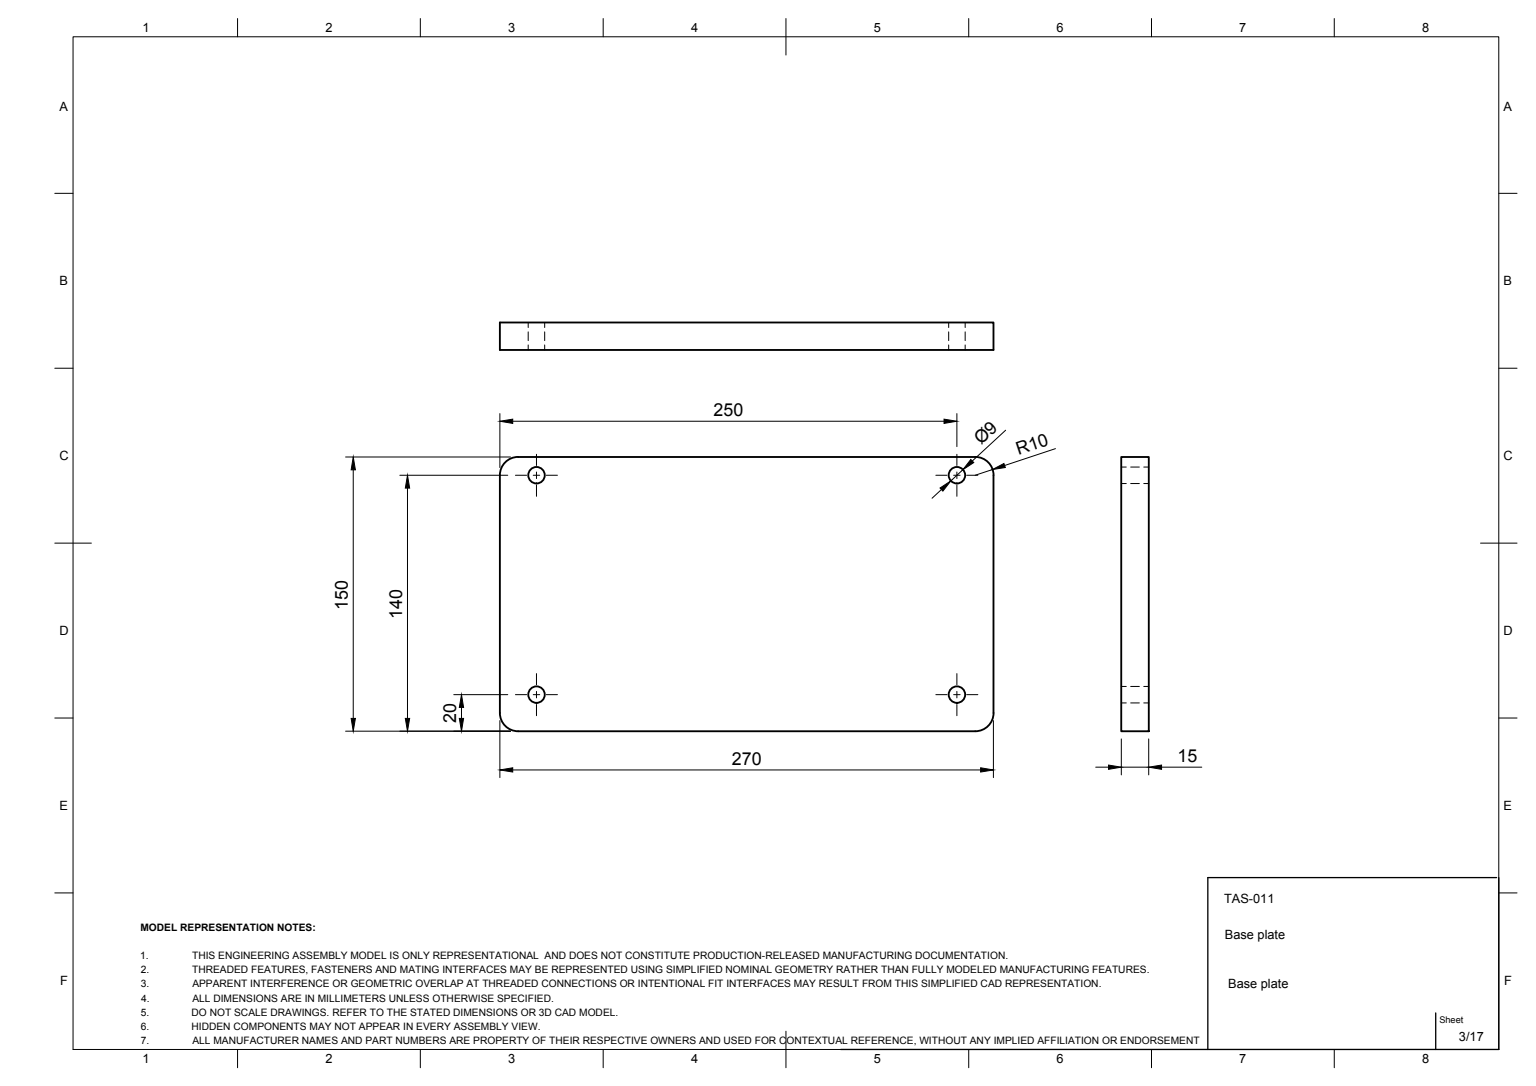
ISO-10303-21;
HEADER;
/* Generated by software containing ST-Developer
 * from STEP Tools, Inc. (www.steptools.com) 
 */

FILE_DESCRIPTION(
/* description */ (
'Independent manual bench leaf bending machine,200mm work width. Fabri
cated welded frame and folding leaf, repeated bushed and fully retaine
d hinge hardware, two handles with bonded grips, beveled clamping beam
 and modeledM12 clamp screws.2mm omitted-workpiece assembly reference 
gap, not a capacity claim. Native135deg hinge travel. Weld sizing, pro
duction fits, material condition, bending capacity, strength and life 
unassigned.'),
/* implementation_level */ '2;1');

FILE_NAME(
/* name */ 'Base plate.step',
/* time_stamp */ '2026-11-14T09:11:34-08:00',
/* author */ (''),
/* organization */ (''),
/* preprocessor_version */ 'ST-DEVELOPER v20.2',
/* originating_system */ 'Autodesk Translation Framework v15.17.0.0',
/* authorisation */ '');

FILE_SCHEMA (('AUTOMOTIVE_DESIGN { 1 0 10303 214 3 1 1 }'));
ENDSEC;

DATA;
#10=MECHANICAL_DESIGN_GEOMETRIC_PRESENTATION_REPRESENTATION('',(#446),#37701);
#410=SHAPE_REPRESENTATION_RELATIONSHIP('SRR','None',#37779,#428);
#428=ADVANCED_BREP_SHAPE_REPRESENTATION('',(#464),#37683);
#446=STYLED_ITEM('',(#37878),#464);
#464=MANIFOLD_SOLID_BREP('Body1',#4144);
#482=FACE_BOUND('',#817,.T.);
#483=FACE_BOUND('',#818,.T.);
#484=FACE_BOUND('',#819,.T.);
#485=FACE_BOUND('',#820,.T.);
#486=FACE_BOUND('',#832,.T.);
#487=FACE_BOUND('',#833,.T.);
#488=FACE_BOUND('',#834,.T.);
#489=FACE_BOUND('',#835,.T.);
#516=PLANE('',#4366);
#517=PLANE('',#4367);
#518=PLANE('',#4377);
#519=PLANE('',#4380);
#520=PLANE('',#4391);
#521=PLANE('',#4392);
#602=FACE_OUTER_BOUND('',#814,.T.);
#603=FACE_OUTER_BOUND('',#815,.T.);
#604=FACE_OUTER_BOUND('',#816,.T.);
#605=FACE_OUTER_BOUND('',#821,.T.);
#606=FACE_OUTER_BOUND('',#822,.T.);
#607=FACE_OUTER_BOUND('',#823,.T.);
#608=FACE_OUTER_BOUND('',#824,.T.);
#609=FACE_OUTER_BOUND('',#825,.T.);
#610=FACE_OUTER_BOUND('',#826,.T.);
#611=FACE_OUTER_BOUND('',#827,.T.);
#612=FACE_OUTER_BOUND('',#828,.T.);
#613=FACE_OUTER_BOUND('',#829,.T.);
#614=FACE_OUTER_BOUND('',#830,.T.);
#615=FACE_OUTER_BOUND('',#831,.T.);
#814=EDGE_LOOP('',(#2639,#2640,#2641,#2642));
#815=EDGE_LOOP('',(#2643,#2644,#2645,#2646));
#816=EDGE_LOOP('',(#2647,#2648,#2649,#2650,#2651,#2652,#2653,#2654));
#817=EDGE_LOOP('',(#2655));
#818=EDGE_LOOP('',(#2656));
#819=EDGE_LOOP('',(#2657));
#820=EDGE_LOOP('',(#2658));
#821=EDGE_LOOP('',(#2659,#2660,#2661,#2662));
#822=EDGE_LOOP('',(#2663,#2664,#2665,#2666));
#823=EDGE_LOOP('',(#2667,#2668,#2669,#2670));
#824=EDGE_LOOP('',(#2671,#2672,#2673,#2674));
#825=EDGE_LOOP('',(#2675,#2676,#2677,#2678));
#826=EDGE_LOOP('',(#2679,#2680,#2681,#2682));
#827=EDGE_LOOP('',(#2683,#2684,#2685,#2686));
#828=EDGE_LOOP('',(#2687,#2688,#2689,#2690));
#829=EDGE_LOOP('',(#2691,#2692,#2693,#2694));
#830=EDGE_LOOP('',(#2695,#2696,#2697,#2698));
#831=EDGE_LOOP('',(#2699,#2700,#2701,#2702,#2703,#2704,#2705,#2706));
#832=EDGE_LOOP('',(#2707));
#833=EDGE_LOOP('',(#2708));
#834=EDGE_LOOP('',(#2709));
#835=EDGE_LOOP('',(#2710));
#1060=LINE('',#5655,#1309);
#1061=LINE('',#5658,#1310);
#1062=LINE('',#5661,#1311);
#1063=LINE('',#5663,#1312);
#1064=LINE('',#5664,#1313);
#1065=LINE('',#5667,#1314);
#1066=LINE('',#5671,#1315);
#1067=LINE('',#5675,#1316);
#1068=LINE('',#5688,#1317);
#1069=LINE('',#5691,#1318);
#1070=LINE('',#5692,#1319);
#1071=LINE('',#5696,#1320);
#1072=LINE('',#5699,#1321);
#1073=LINE('',#5700,#1322);
#1074=LINE('',#5704,#1323);
#1075=LINE('',#5708,#1324);
#1076=LINE('',#5712,#1325);
#1077=LINE('',#5716,#1326);
#1078=LINE('',#5720,#1327);
#1079=LINE('',#5722,#1328);
#1309=VECTOR('',#4715,10.);
#1310=VECTOR('',#4718,10.);
#1311=VECTOR('',#4721,10.);
#1312=VECTOR('',#4722,10.);
#1313=VECTOR('',#4723,10.);
#1314=VECTOR('',#4726,10.);
#1315=VECTOR('',#4729,10.);
#1316=VECTOR('',#4732,10.);
#1317=VECTOR('',#4747,10.);
#1318=VECTOR('',#4750,10.);
#1319=VECTOR('',#4751,10.);
#1320=VECTOR('',#4756,10.);
#1321=VECTOR('',#4759,10.);
#1322=VECTOR('',#4760,10.);
#1323=VECTOR('',#4765,10.);
#1324=VECTOR('',#4770,4.5);
#1325=VECTOR('',#4775,4.5);
#1326=VECTOR('',#4780,4.5);
#1327=VECTOR('',#4785,4.5);
#1328=VECTOR('',#4788,10.);
#1558=CIRCLE('',#4364,10.);
#1559=CIRCLE('',#4365,10.);
#1560=CIRCLE('',#4368,10.);
#1561=CIRCLE('',#4369,10.);
#1562=CIRCLE('',#4370,10.);
#1563=CIRCLE('',#4371,4.5);
#1564=CIRCLE('',#4372,4.5);
#1565=CIRCLE('',#4373,4.5);
#1566=CIRCLE('',#4374,4.5);
#1567=CIRCLE('',#4376,10.);
#1568=CIRCLE('',#4379,10.);
#1569=CIRCLE('',#4382,10.);
#1570=CIRCLE('',#4384,4.5);
#1571=CIRCLE('',#4386,4.5);
#1572=CIRCLE('',#4388,4.5);
#1573=CIRCLE('',#4390,4.5);
#1637=VERTEX_POINT('',#5651);
#1638=VERTEX_POINT('',#5652);
#1639=VERTEX_POINT('',#5654);
#1640=VERTEX_POINT('',#5656);
#1641=VERTEX_POINT('',#5660);
#1642=VERTEX_POINT('',#5662);
#1643=VERTEX_POINT('',#5666);
#1644=VERTEX_POINT('',#5668);
#1645=VERTEX_POINT('',#5670);
#1646=VERTEX_POINT('',#5672);
#1647=VERTEX_POINT('',#5674);
#1648=VERTEX_POINT('',#5677);
#1649=VERTEX_POINT('',#5679);
#1650=VERTEX_POINT('',#5681);
#1651=VERTEX_POINT('',#5683);
#1652=VERTEX_POINT('',#5686);
#1653=VERTEX_POINT('',#5690);
#1654=VERTEX_POINT('',#5694);
#1655=VERTEX_POINT('',#5698);
#1656=VERTEX_POINT('',#5702);
#1657=VERTEX_POINT('',#5706);
#1658=VERTEX_POINT('',#5710);
#1659=VERTEX_POINT('',#5714);
#1660=VERTEX_POINT('',#5718);
#2053=EDGE_CURVE('',#1637,#1638,#1558,.T.);
#2054=EDGE_CURVE('',#1638,#1639,#1060,.T.);
#2055=EDGE_CURVE('',#1639,#1640,#1559,.T.);
#2056=EDGE_CURVE('',#1640,#1637,#1061,.T.);
#2057=EDGE_CURVE('',#1640,#1641,#1062,.F.);
#2058=EDGE_CURVE('',#1642,#1641,#1063,.T.);
#2059=EDGE_CURVE('',#1637,#1642,#1064,.F.);
#2060=EDGE_CURVE('',#1643,#1639,#1065,.F.);
#2061=EDGE_CURVE('',#1644,#1643,#1560,.T.);
#2062=EDGE_CURVE('',#1645,#1644,#1066,.F.);
#2063=EDGE_CURVE('',#1646,#1645,#1561,.T.);
#2064=EDGE_CURVE('',#1647,#1646,#1067,.F.);
#2065=EDGE_CURVE('',#1641,#1647,#1562,.T.);
#2066=EDGE_CURVE('',#1648,#1648,#1563,.T.);
#2067=EDGE_CURVE('',#1649,#1649,#1564,.T.);
#2068=EDGE_CURVE('',#1650,#1650,#1565,.T.);
#2069=EDGE_CURVE('',#1651,#1651,#1566,.T.);
#2070=EDGE_CURVE('',#1652,#1642,#1567,.T.);
#2071=EDGE_CURVE('',#1647,#1652,#1068,.T.);
#2072=EDGE_CURVE('',#1653,#1646,#1069,.T.);
#2073=EDGE_CURVE('',#1652,#1653,#1070,.F.);
#2074=EDGE_CURVE('',#1654,#1653,#1568,.T.);
#2075=EDGE_CURVE('',#1645,#1654,#1071,.T.);
#2076=EDGE_CURVE('',#1655,#1644,#1072,.T.);
#2077=EDGE_CURVE('',#1654,#1655,#1073,.F.);
#2078=EDGE_CURVE('',#1656,#1655,#1569,.T.);
#2079=EDGE_CURVE('',#1643,#1656,#1074,.T.);
#2080=EDGE_CURVE('',#1657,#1657,#1570,.T.);
#2081=EDGE_CURVE('',#1657,#1648,#1075,.T.);
#2082=EDGE_CURVE('',#1658,#1658,#1571,.T.);
#2083=EDGE_CURVE('',#1658,#1649,#1076,.T.);
#2084=EDGE_CURVE('',#1659,#1659,#1572,.T.);
#2085=EDGE_CURVE('',#1659,#1650,#1077,.T.);
#2086=EDGE_CURVE('',#1660,#1660,#1573,.T.);
#2087=EDGE_CURVE('',#1660,#1651,#1078,.T.);
#2088=EDGE_CURVE('',#1656,#1638,#1079,.F.);
#2639=ORIENTED_EDGE('',*,*,#2053,.T.);
#2640=ORIENTED_EDGE('',*,*,#2054,.T.);
#2641=ORIENTED_EDGE('',*,*,#2055,.T.);
#2642=ORIENTED_EDGE('',*,*,#2056,.T.);
#2643=ORIENTED_EDGE('',*,*,#2056,.F.);
#2644=ORIENTED_EDGE('',*,*,#2057,.T.);
#2645=ORIENTED_EDGE('',*,*,#2058,.F.);
#2646=ORIENTED_EDGE('',*,*,#2059,.F.);
#2647=ORIENTED_EDGE('',*,*,#2055,.F.);
#2648=ORIENTED_EDGE('',*,*,#2060,.F.);
#2649=ORIENTED_EDGE('',*,*,#2061,.F.);
#2650=ORIENTED_EDGE('',*,*,#2062,.F.);
#2651=ORIENTED_EDGE('',*,*,#2063,.F.);
#2652=ORIENTED_EDGE('',*,*,#2064,.F.);
#2653=ORIENTED_EDGE('',*,*,#2065,.F.);
#2654=ORIENTED_EDGE('',*,*,#2057,.F.);
#2655=ORIENTED_EDGE('',*,*,#2066,.T.);
#2656=ORIENTED_EDGE('',*,*,#2067,.T.);
#2657=ORIENTED_EDGE('',*,*,#2068,.T.);
#2658=ORIENTED_EDGE('',*,*,#2069,.T.);
#2659=ORIENTED_EDGE('',*,*,#2070,.T.);
#2660=ORIENTED_EDGE('',*,*,#2058,.T.);
#2661=ORIENTED_EDGE('',*,*,#2065,.T.);
#2662=ORIENTED_EDGE('',*,*,#2071,.T.);
#2663=ORIENTED_EDGE('',*,*,#2071,.F.);
#2664=ORIENTED_EDGE('',*,*,#2064,.T.);
#2665=ORIENTED_EDGE('',*,*,#2072,.F.);
#2666=ORIENTED_EDGE('',*,*,#2073,.F.);
#2667=ORIENTED_EDGE('',*,*,#2074,.T.);
#2668=ORIENTED_EDGE('',*,*,#2072,.T.);
#2669=ORIENTED_EDGE('',*,*,#2063,.T.);
#2670=ORIENTED_EDGE('',*,*,#2075,.T.);
#2671=ORIENTED_EDGE('',*,*,#2075,.F.);
#2672=ORIENTED_EDGE('',*,*,#2062,.T.);
#2673=ORIENTED_EDGE('',*,*,#2076,.F.);
#2674=ORIENTED_EDGE('',*,*,#2077,.F.);
#2675=ORIENTED_EDGE('',*,*,#2078,.T.);
#2676=ORIENTED_EDGE('',*,*,#2076,.T.);
#2677=ORIENTED_EDGE('',*,*,#2061,.T.);
#2678=ORIENTED_EDGE('',*,*,#2079,.T.);
#2679=ORIENTED_EDGE('',*,*,#2080,.F.);
#2680=ORIENTED_EDGE('',*,*,#2081,.T.);
#2681=ORIENTED_EDGE('',*,*,#2066,.F.);
#2682=ORIENTED_EDGE('',*,*,#2081,.F.);
#2683=ORIENTED_EDGE('',*,*,#2082,.F.);
#2684=ORIENTED_EDGE('',*,*,#2083,.T.);
#2685=ORIENTED_EDGE('',*,*,#2067,.F.);
#2686=ORIENTED_EDGE('',*,*,#2083,.F.);
#2687=ORIENTED_EDGE('',*,*,#2084,.F.);
#2688=ORIENTED_EDGE('',*,*,#2085,.T.);
#2689=ORIENTED_EDGE('',*,*,#2068,.F.);
#2690=ORIENTED_EDGE('',*,*,#2085,.F.);
#2691=ORIENTED_EDGE('',*,*,#2086,.F.);
#2692=ORIENTED_EDGE('',*,*,#2087,.T.);
#2693=ORIENTED_EDGE('',*,*,#2069,.F.);
#2694=ORIENTED_EDGE('',*,*,#2087,.F.);
#2695=ORIENTED_EDGE('',*,*,#2054,.F.);
#2696=ORIENTED_EDGE('',*,*,#2088,.F.);
#2697=ORIENTED_EDGE('',*,*,#2079,.F.);
#2698=ORIENTED_EDGE('',*,*,#2060,.T.);
#2699=ORIENTED_EDGE('',*,*,#2053,.F.);
#2700=ORIENTED_EDGE('',*,*,#2059,.T.);
#2701=ORIENTED_EDGE('',*,*,#2070,.F.);
#2702=ORIENTED_EDGE('',*,*,#2073,.T.);
#2703=ORIENTED_EDGE('',*,*,#2074,.F.);
#2704=ORIENTED_EDGE('',*,*,#2077,.T.);
#2705=ORIENTED_EDGE('',*,*,#2078,.F.);
#2706=ORIENTED_EDGE('',*,*,#2088,.T.);
#2707=ORIENTED_EDGE('',*,*,#2080,.T.);
#2708=ORIENTED_EDGE('',*,*,#2082,.T.);
#2709=ORIENTED_EDGE('',*,*,#2084,.T.);
#2710=ORIENTED_EDGE('',*,*,#2086,.T.);
#3811=CYLINDRICAL_SURFACE('',#4363,10.);
#3812=CYLINDRICAL_SURFACE('',#4375,10.);
#3813=CYLINDRICAL_SURFACE('',#4378,10.);
#3814=CYLINDRICAL_SURFACE('',#4381,10.);
#3815=CYLINDRICAL_SURFACE('',#4383,4.5);
#3816=CYLINDRICAL_SURFACE('',#4385,4.5);
#3817=CYLINDRICAL_SURFACE('',#4387,4.5);
#3818=CYLINDRICAL_SURFACE('',#4389,4.5);
#3932=ADVANCED_FACE('',(#602),#3811,.T.);
#3933=ADVANCED_FACE('',(#603),#516,.T.);
#3934=ADVANCED_FACE('',(#604,#482,#483,#484,#485),#517,.F.);
#3935=ADVANCED_FACE('',(#605),#3812,.T.);
#3936=ADVANCED_FACE('',(#606),#518,.T.);
#3937=ADVANCED_FACE('',(#607),#3813,.T.);
#3938=ADVANCED_FACE('',(#608),#519,.T.);
#3939=ADVANCED_FACE('',(#609),#3814,.T.);
#3940=ADVANCED_FACE('',(#610),#3815,.F.);
#3941=ADVANCED_FACE('',(#611),#3816,.F.);
#3942=ADVANCED_FACE('',(#612),#3817,.F.);
#3943=ADVANCED_FACE('',(#613),#3818,.F.);
#3944=ADVANCED_FACE('',(#614),#520,.T.);
#3945=ADVANCED_FACE('',(#615,#486,#487,#488,#489),#521,.T.);
#4144=CLOSED_SHELL('',(#3932,#3933,#3934,#3935,#3936,#3937,#3938,#3939,
#3940,#3941,#3942,#3943,#3944,#3945));
#4362=AXIS2_PLACEMENT_3D('',#5649,#4709,#4710);
#4363=AXIS2_PLACEMENT_3D('',#5650,#4711,#4712);
#4364=AXIS2_PLACEMENT_3D('',#5653,#4713,#4714);
#4365=AXIS2_PLACEMENT_3D('',#5657,#4716,#4717);
#4366=AXIS2_PLACEMENT_3D('',#5659,#4719,#4720);
#4367=AXIS2_PLACEMENT_3D('',#5665,#4724,#4725);
#4368=AXIS2_PLACEMENT_3D('',#5669,#4727,#4728);
#4369=AXIS2_PLACEMENT_3D('',#5673,#4730,#4731);
#4370=AXIS2_PLACEMENT_3D('',#5676,#4733,#4734);
#4371=AXIS2_PLACEMENT_3D('',#5678,#4735,#4736);
#4372=AXIS2_PLACEMENT_3D('',#5680,#4737,#4738);
#4373=AXIS2_PLACEMENT_3D('',#5682,#4739,#4740);
#4374=AXIS2_PLACEMENT_3D('',#5684,#4741,#4742);
#4375=AXIS2_PLACEMENT_3D('',#5685,#4743,#4744);
#4376=AXIS2_PLACEMENT_3D('',#5687,#4745,#4746);
#4377=AXIS2_PLACEMENT_3D('',#5689,#4748,#4749);
#4378=AXIS2_PLACEMENT_3D('',#5693,#4752,#4753);
#4379=AXIS2_PLACEMENT_3D('',#5695,#4754,#4755);
#4380=AXIS2_PLACEMENT_3D('',#5697,#4757,#4758);
#4381=AXIS2_PLACEMENT_3D('',#5701,#4761,#4762);
#4382=AXIS2_PLACEMENT_3D('',#5703,#4763,#4764);
#4383=AXIS2_PLACEMENT_3D('',#5705,#4766,#4767);
#4384=AXIS2_PLACEMENT_3D('',#5707,#4768,#4769);
#4385=AXIS2_PLACEMENT_3D('',#5709,#4771,#4772);
#4386=AXIS2_PLACEMENT_3D('',#5711,#4773,#4774);
#4387=AXIS2_PLACEMENT_3D('',#5713,#4776,#4777);
#4388=AXIS2_PLACEMENT_3D('',#5715,#4778,#4779);
#4389=AXIS2_PLACEMENT_3D('',#5717,#4781,#4782);
#4390=AXIS2_PLACEMENT_3D('',#5719,#4783,#4784);
#4391=AXIS2_PLACEMENT_3D('',#5721,#4786,#4787);
#4392=AXIS2_PLACEMENT_3D('',#5723,#4789,#4790);
#4709=DIRECTION('axis',(0.,0.,1.));
#4710=DIRECTION('refdir',(1.,0.,0.));
#4711=DIRECTION('center_axis',(0.,0.,1.));
#4712=DIRECTION('ref_axis',(0.707106781186548,0.707106781186548,0.));
#4713=DIRECTION('center_axis',(0.,0.,-1.));
#4714=DIRECTION('ref_axis',(0.707106781186548,0.707106781186548,0.));
#4715=DIRECTION('',(0.,0.,-1.));
#4716=DIRECTION('center_axis',(0.,0.,1.));
#4717=DIRECTION('ref_axis',(0.707106781186548,0.707106781186548,0.));
#4718=DIRECTION('',(0.,0.,1.));
#4719=DIRECTION('center_axis',(0.,1.,0.));
#4720=DIRECTION('ref_axis',(-1.,0.,0.));
#4721=DIRECTION('',(1.,0.,0.));
#4722=DIRECTION('',(0.,0.,-1.));
#4723=DIRECTION('',(1.,0.,0.));
#4724=DIRECTION('center_axis',(0.,0.,1.));
#4725=DIRECTION('ref_axis',(1.,0.,0.));
#4726=DIRECTION('',(0.,-1.,0.));
#4727=DIRECTION('center_axis',(0.,0.,1.));
#4728=DIRECTION('ref_axis',(0.707106781186548,-0.707106781186548,0.));
#4729=DIRECTION('',(-1.,0.,0.));
#4730=DIRECTION('center_axis',(0.,0.,1.));
#4731=DIRECTION('ref_axis',(-0.707106781186548,-0.707106781186548,0.));
#4732=DIRECTION('',(0.,1.,0.));
#4733=DIRECTION('center_axis',(0.,0.,1.));
#4734=DIRECTION('ref_axis',(-0.707106781186548,0.707106781186548,0.));
#4735=DIRECTION('center_axis',(0.,0.,1.));
#4736=DIRECTION('ref_axis',(1.,0.,0.));
#4737=DIRECTION('center_axis',(0.,0.,1.));
#4738=DIRECTION('ref_axis',(1.,0.,0.));
#4739=DIRECTION('center_axis',(0.,0.,1.));
#4740=DIRECTION('ref_axis',(1.,0.,0.));
#4741=DIRECTION('center_axis',(0.,0.,1.));
#4742=DIRECTION('ref_axis',(1.,0.,0.));
#4743=DIRECTION('center_axis',(0.,0.,1.));
#4744=DIRECTION('ref_axis',(-0.707106781186548,0.707106781186548,0.));
#4745=DIRECTION('center_axis',(0.,0.,-1.));
#4746=DIRECTION('ref_axis',(-0.707106781186548,0.707106781186548,0.));
#4747=DIRECTION('',(0.,0.,1.));
#4748=DIRECTION('center_axis',(-1.,0.,0.));
#4749=DIRECTION('ref_axis',(0.,-1.,0.));
#4750=DIRECTION('',(0.,0.,-1.));
#4751=DIRECTION('',(0.,1.,0.));
#4752=DIRECTION('center_axis',(0.,0.,1.));
#4753=DIRECTION('ref_axis',(-0.707106781186548,-0.707106781186548,0.));
#4754=DIRECTION('center_axis',(0.,0.,-1.));
#4755=DIRECTION('ref_axis',(-0.707106781186548,-0.707106781186548,0.));
#4756=DIRECTION('',(0.,0.,1.));
#4757=DIRECTION('center_axis',(0.,-1.,0.));
#4758=DIRECTION('ref_axis',(1.,0.,0.));
#4759=DIRECTION('',(0.,0.,-1.));
#4760=DIRECTION('',(-1.,0.,0.));
#4761=DIRECTION('center_axis',(0.,0.,1.));
#4762=DIRECTION('ref_axis',(0.707106781186548,-0.707106781186548,0.));
#4763=DIRECTION('center_axis',(0.,0.,-1.));
#4764=DIRECTION('ref_axis',(0.707106781186548,-0.707106781186548,0.));
#4765=DIRECTION('',(0.,0.,1.));
#4766=DIRECTION('center_axis',(0.,0.,-1.));
#4767=DIRECTION('ref_axis',(1.,0.,0.));
#4768=DIRECTION('center_axis',(0.,0.,-1.));
#4769=DIRECTION('ref_axis',(1.,0.,0.));
#4770=DIRECTION('',(0.,0.,-1.));
#4771=DIRECTION('center_axis',(0.,0.,-1.));
#4772=DIRECTION('ref_axis',(1.,0.,0.));
#4773=DIRECTION('center_axis',(0.,0.,-1.));
#4774=DIRECTION('ref_axis',(1.,0.,0.));
#4775=DIRECTION('',(0.,0.,-1.));
#4776=DIRECTION('center_axis',(0.,0.,-1.));
#4777=DIRECTION('ref_axis',(1.,0.,0.));
#4778=DIRECTION('center_axis',(0.,0.,-1.));
#4779=DIRECTION('ref_axis',(1.,0.,0.));
#4780=DIRECTION('',(0.,0.,-1.));
#4781=DIRECTION('center_axis',(0.,0.,-1.));
#4782=DIRECTION('ref_axis',(1.,0.,0.));
#4783=DIRECTION('center_axis',(0.,0.,-1.));
#4784=DIRECTION('ref_axis',(1.,0.,0.));
#4785=DIRECTION('',(0.,0.,-1.));
#4786=DIRECTION('center_axis',(1.,0.,0.));
#4787=DIRECTION('ref_axis',(0.,1.,0.));
#4788=DIRECTION('',(0.,-1.,0.));
#4789=DIRECTION('center_axis',(0.,0.,1.));
#4790=DIRECTION('ref_axis',(1.,0.,0.));
#5649=CARTESIAN_POINT('',(0.,0.,0.));
#5650=CARTESIAN_POINT('Origin',(25.,125.,0.));
#5651=CARTESIAN_POINT('',(25.,135.,10.));
#5652=CARTESIAN_POINT('',(35.,125.,10.));
#5653=CARTESIAN_POINT('Origin',(25.,125.,10.));
#5654=CARTESIAN_POINT('',(35.,125.,-5.));
#5655=CARTESIAN_POINT('',(35.,125.,0.));
#5656=CARTESIAN_POINT('',(25.,135.,-5.));
#5657=CARTESIAN_POINT('Origin',(25.,125.,-5.));
#5658=CARTESIAN_POINT('',(25.,135.,0.));
#5659=CARTESIAN_POINT('Origin',(40.,135.,0.));
#5660=CARTESIAN_POINT('',(-105.,135.,-5.));
#5661=CARTESIAN_POINT('',(2.5,135.,-5.));
#5662=CARTESIAN_POINT('',(-105.,135.,10.));
#5663=CARTESIAN_POINT('',(-105.,135.,0.));
#5664=CARTESIAN_POINT('',(2.5,135.,10.));
#5665=CARTESIAN_POINT('Origin',(-35.,0.,-5.));
#5666=CARTESIAN_POINT('',(35.,-125.,-5.));
#5667=CARTESIAN_POINT('',(35.,-65.,-5.));
#5668=CARTESIAN_POINT('',(25.,-135.,-5.));
#5669=CARTESIAN_POINT('Origin',(25.,-125.,-5.));
#5670=CARTESIAN_POINT('',(-105.,-135.,-5.));
#5671=CARTESIAN_POINT('',(-72.5,-135.,-5.));
#5672=CARTESIAN_POINT('',(-115.,-125.,-5.));
#5673=CARTESIAN_POINT('Origin',(-105.,-125.,-5.));
#5674=CARTESIAN_POINT('',(-115.,125.,-5.));
#5675=CARTESIAN_POINT('',(-115.,65.,-5.));
#5676=CARTESIAN_POINT('Origin',(-105.,125.,-5.));
#5677=CARTESIAN_POINT('',(20.5,-115.,-5.));
#5678=CARTESIAN_POINT('Origin',(25.,-115.,-5.));
#5679=CARTESIAN_POINT('',(-99.5,-115.,-5.));
#5680=CARTESIAN_POINT('Origin',(-95.,-115.,-5.));
#5681=CARTESIAN_POINT('',(-99.5,115.,-5.));
#5682=CARTESIAN_POINT('Origin',(-95.,115.,-5.));
#5683=CARTESIAN_POINT('',(20.5,115.,-5.));
#5684=CARTESIAN_POINT('Origin',(25.,115.,-5.));
#5685=CARTESIAN_POINT('Origin',(-105.,125.,0.));
#5686=CARTESIAN_POINT('',(-115.,125.,10.));
#5687=CARTESIAN_POINT('Origin',(-105.,125.,10.));
#5688=CARTESIAN_POINT('',(-115.,125.,0.));
#5689=CARTESIAN_POINT('Origin',(-115.,130.,0.));
#5690=CARTESIAN_POINT('',(-115.,-125.,10.));
#5691=CARTESIAN_POINT('',(-115.,-125.,0.));
#5692=CARTESIAN_POINT('',(-115.,65.,10.));
#5693=CARTESIAN_POINT('Origin',(-105.,-125.,0.));
#5694=CARTESIAN_POINT('',(-105.,-135.,10.));
#5695=CARTESIAN_POINT('Origin',(-105.,-125.,10.));
#5696=CARTESIAN_POINT('',(-105.,-135.,0.));
#5697=CARTESIAN_POINT('Origin',(-110.,-135.,0.));
#5698=CARTESIAN_POINT('',(25.,-135.,10.));
#5699=CARTESIAN_POINT('',(25.,-135.,0.));
#5700=CARTESIAN_POINT('',(-72.5,-135.,10.));
#5701=CARTESIAN_POINT('Origin',(25.,-125.,0.));
#5702=CARTESIAN_POINT('',(35.,-125.,10.));
#5703=CARTESIAN_POINT('Origin',(25.,-125.,10.));
#5704=CARTESIAN_POINT('',(35.,-125.,0.));
#5705=CARTESIAN_POINT('Origin',(25.,-115.,5.));
#5706=CARTESIAN_POINT('',(20.5,-115.,10.));
#5707=CARTESIAN_POINT('Origin',(25.,-115.,10.));
#5708=CARTESIAN_POINT('',(20.5,-115.,5.));
#5709=CARTESIAN_POINT('Origin',(-95.,-115.,5.));
#5710=CARTESIAN_POINT('',(-99.5,-115.,10.));
#5711=CARTESIAN_POINT('Origin',(-95.,-115.,10.));
#5712=CARTESIAN_POINT('',(-99.5,-115.,5.));
#5713=CARTESIAN_POINT('Origin',(-95.,115.,5.));
#5714=CARTESIAN_POINT('',(-99.5,115.,10.));
#5715=CARTESIAN_POINT('Origin',(-95.,115.,10.));
#5716=CARTESIAN_POINT('',(-99.5,115.,5.));
#5717=CARTESIAN_POINT('Origin',(25.,115.,5.));
#5718=CARTESIAN_POINT('',(20.5,115.,10.));
#5719=CARTESIAN_POINT('Origin',(25.,115.,10.));
#5720=CARTESIAN_POINT('',(20.5,115.,5.));
#5721=CARTESIAN_POINT('Origin',(35.,-130.,0.));
#5722=CARTESIAN_POINT('',(35.,-65.,10.));
#5723=CARTESIAN_POINT('Origin',(-35.,0.,10.));
#37663=UNCERTAINTY_MEASURE_WITH_UNIT(LENGTH_MEASURE(0.01),#37702,
'DISTANCE_ACCURACY_VALUE',
'Maximum model space distance between geometric entities at asserted c
onnectivities');
#37681=UNCERTAINTY_MEASURE_WITH_UNIT(LENGTH_MEASURE(0.01),#37702,
'DISTANCE_ACCURACY_VALUE',
'Maximum model space distance between geometric entities at asserted c
onnectivities');
#37683=(
GEOMETRIC_REPRESENTATION_CONTEXT(3)
GLOBAL_UNCERTAINTY_ASSIGNED_CONTEXT((#37663))
GLOBAL_UNIT_ASSIGNED_CONTEXT((#37702,#37704,#37705))
REPRESENTATION_CONTEXT('','3D')
);
#37701=(
GEOMETRIC_REPRESENTATION_CONTEXT(3)
GLOBAL_UNCERTAINTY_ASSIGNED_CONTEXT((#37681))
GLOBAL_UNIT_ASSIGNED_CONTEXT((#37702,#37704,#37705))
REPRESENTATION_CONTEXT('','3D')
);
#37702=(
LENGTH_UNIT()
NAMED_UNIT(*)
SI_UNIT(.MILLI.,.METRE.)
);
#37704=(
NAMED_UNIT(*)
PLANE_ANGLE_UNIT()
SI_UNIT($,.RADIAN.)
);
#37705=(
NAMED_UNIT(*)
SI_UNIT($,.STERADIAN.)
SOLID_ANGLE_UNIT()
);
#37707=SHAPE_DEFINITION_REPRESENTATION(#37726,#37779);
#37726=PRODUCT_DEFINITION_SHAPE('',$,#37799);
#37779=SHAPE_REPRESENTATION('',(#4362),#37683);
#37797=PRODUCT_DEFINITION_CONTEXT('part definition',#37856,'design');
#37799=PRODUCT_DEFINITION('Base plate','Base plate',#37818,#37797);
#37818=PRODUCT_DEFINITION_FORMATION('',$,#37859);
#37856=APPLICATION_CONTEXT(
'Core Data for Automotive Mechanical Design Process');
#37857=PRODUCT_CONTEXT('part definition',#37856,'mechanical');
#37859=PRODUCT('Base plate','Base plate','Base plate',(#37857));
#37878=PRESENTATION_STYLE_ASSIGNMENT((#37886));
#37886=SURFACE_STYLE_USAGE(.BOTH.,#37894);
#37894=SURFACE_SIDE_STYLE('',(#37902));
#37902=SURFACE_STYLE_FILL_AREA(#37910);
#37910=FILL_AREA_STYLE('Opaque(23,69,131)',(#37918));
#37918=FILL_AREA_STYLE_COLOUR('Opaque(23,69,131)',#37926);
#37926=COLOUR_RGB('Opaque(23,69,131)',0.0901960784313725,0.270588235294118,
0.513725490196078);
ENDSEC;
END-ISO-10303-21;
